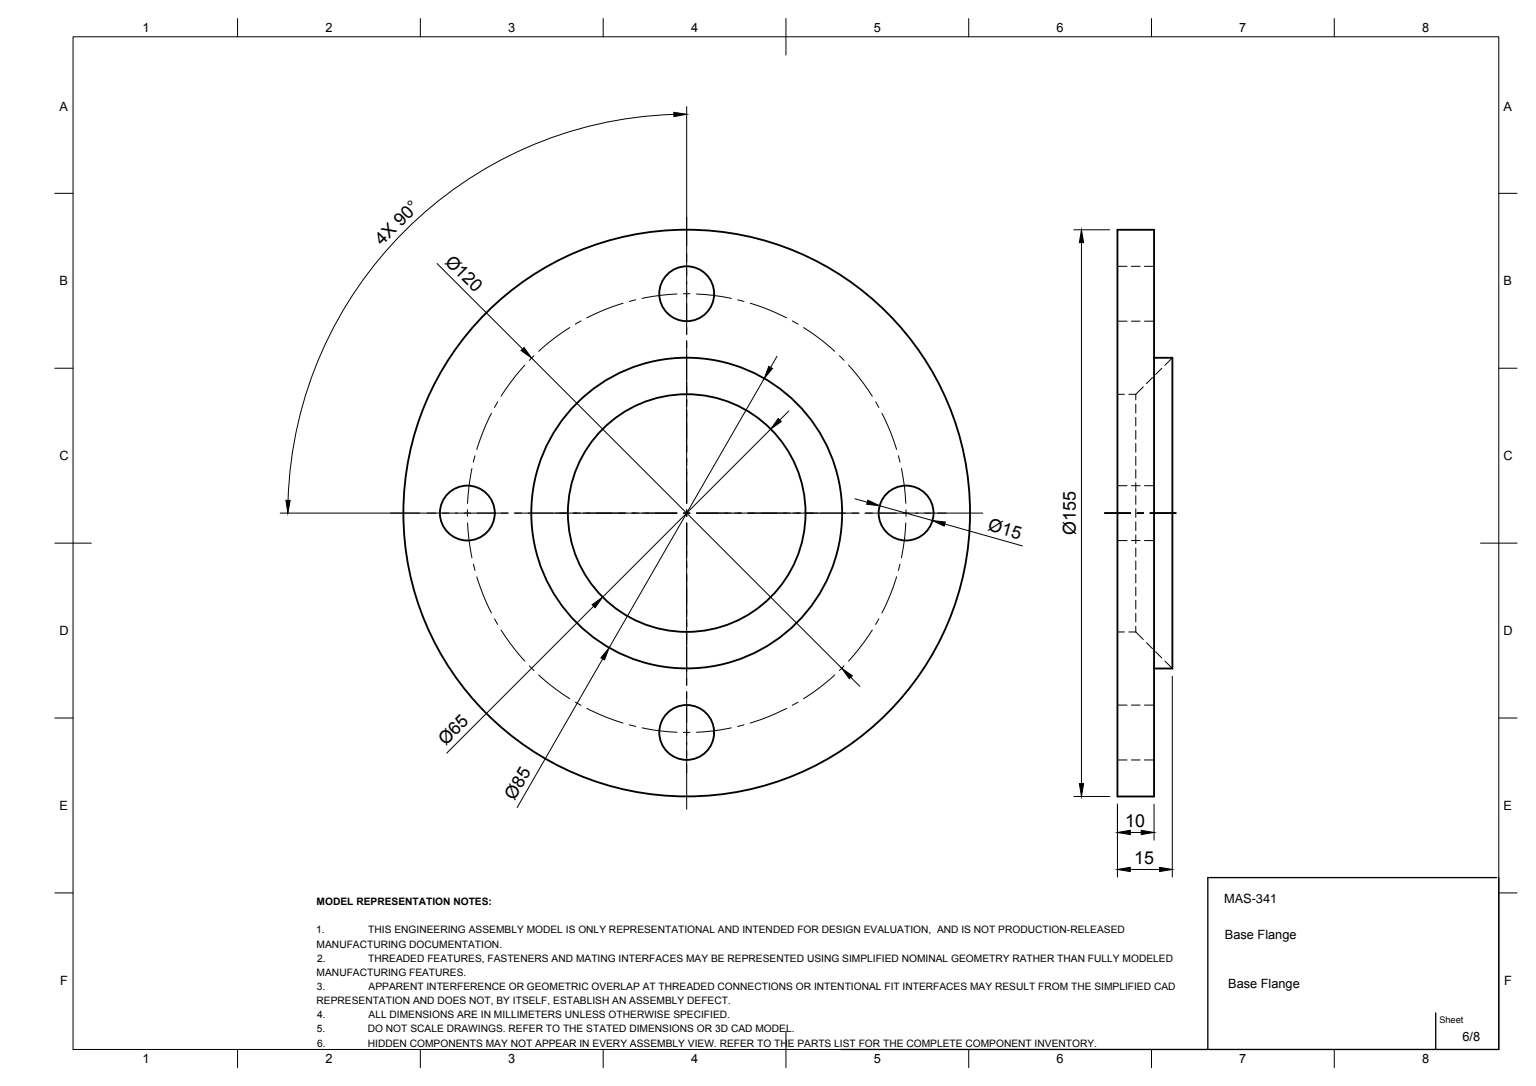
ISO-10303-21;
HEADER;
FILE_DESCRIPTION (('STEP AP214'),
    '1' );
FILE_NAME ('Base Flange.step',
    '2026-10-08T00:39:10',
    ( '' ),
    ( '' ),
    'SwSTEP 2.0',
    'SolidWorks 2025',
    '' );
FILE_SCHEMA (( 'AUTOMOTIVE_DESIGN' ));
ENDSEC;

DATA;
#35=DIRECTION ( 'NONE',  ( -0.000000000000000000, -0.000000000000000000, 1.000000000000000000 ) ) ;
#98=VERTEX_POINT ( 'NONE', #17267 ) ;
#119=ORIENTED_EDGE ( 'NONE', *, *, #13238, .T. ) ;
#143=CIRCLE ( 'NONE', #11572, 77.50000000000000000 ) ;
#167=ORIENTED_EDGE ( 'NONE', *, *, #19754, .F. ) ;
#188=( GEOMETRIC_REPRESENTATION_CONTEXT ( 3 ) GLOBAL_UNCERTAINTY_ASSIGNED_CONTEXT ( ( #9055 ) ) GLOBAL_UNIT_ASSIGNED_CONTEXT ( ( #6659, #405, #9614 ) ) REPRESENTATION_CONTEXT ( 'NONE', 'WORKASPACE' ) );
#215=ORIENTED_EDGE ( 'NONE', *, *, #14623, .F. ) ;
#270=VERTEX_POINT ( 'NONE', #10443 ) ;
#322=EDGE_LOOP ( 'NONE', ( #19155, #18434, #14933, #18302 ) ) ;
#335=DIRECTION ( 'NONE',  ( -0.000000000000000000, -0.000000000000000000, 1.000000000000000000 ) ) ;
#336=DIRECTION ( 'NONE',  ( -0.000000000000000000, -0.000000000000000000, 1.000000000000000000 ) ) ;
#359=CARTESIAN_POINT ( 'NONE',  ( 0.000000000000000000, 0.000000000000000000, -110.0000000000000000 ) ) ;
#405=( NAMED_UNIT ( * ) PLANE_ANGLE_UNIT ( ) SI_UNIT ( $, .RADIAN. ) );
#414=DIRECTION ( 'NONE',  ( 1.000000000000000000, 0.000000000000000000, 0.000000000000000000 ) ) ;
#420=AXIS2_PLACEMENT_3D ( 'NONE', #20059, #15147, #19952 ) ;
#423=CYLINDRICAL_SURFACE ( 'NONE', #14783, 77.50000000000000000 ) ;
#435=DIRECTION ( 'NONE',  ( -1.000000000000000000, 0.000000000000000000, 0.000000000000000000 ) ) ;
#443=CARTESIAN_POINT ( 'NONE',  ( 52.50000000000000711, 6.293851260911244545E-13, -115.0000000000000000 ) ) ;
#482=DIRECTION ( 'NONE',  ( 1.000000000000000000, 0.000000000000000000, 0.000000000000000000 ) ) ;
#529=ORIENTED_EDGE ( 'NONE', *, *, #2169, .T. ) ;
#557=VECTOR ( 'NONE', #16246, 1000.000000000000000 ) ;
#598=VECTOR ( 'NONE', #5827, 1000.000000000000000 ) ;
#610=AXIS2_PLACEMENT_3D ( 'NONE', #18415, #15333, #2864 ) ;
#800=FACE_OUTER_BOUND ( 'NONE', #13112, .T. ) ;
#839=ORIENTED_EDGE ( 'NONE', *, *, #18273, .F. ) ;
#840=ORIENTED_EDGE ( 'NONE', *, *, #17283, .T. ) ;
#862=CLOSED_SHELL ( 'NONE', ( #17922, #12414, #11863, #7855, #11249, #16008, #19643, #18744, #7325, #8273, #4630, #7416, #13850, #8626, #3371, #2282, #10782, #5475 ) ) ;
#1012=EDGE_LOOP ( 'NONE', ( #5410, #2459 ) ) ;
#1023=DIRECTION ( 'NONE',  ( -0.000000000000000000, -0.000000000000000000, 1.000000000000000000 ) ) ;
#1072=FACE_OUTER_BOUND ( 'NONE', #19255, .T. ) ;
#1123=EDGE_CURVE ( 'NONE', #2923, #13175, #17579, .T. ) ;
#1126=CARTESIAN_POINT ( 'NONE',  ( 7.500000000000420997, -60.00000000000000000, -115.0000000000000000 ) ) ;
#1215=AXIS2_PLACEMENT_3D ( 'NONE', #17388, #3363, #5010 ) ;
#1231=DIRECTION ( 'NONE',  ( 0.000000000000000000, 0.000000000000000000, -1.000000000000000000 ) ) ;
#1240=SHAPE_REPRESENTATION_RELATIONSHIP ( 'NONE' , 'NONE' ,  #6269, #19668 ) ;
#1250=FACE_OUTER_BOUND ( 'NONE', #9273, .T. ) ;
#1270=VERTEX_POINT ( 'NONE', #8648 ) ;
#1387=CARTESIAN_POINT ( 'NONE',  ( 60.00000000000000711, 6.284666409917639535E-13, -115.0000000000000000 ) ) ;
#1398=CARTESIAN_POINT ( 'NONE',  ( -42.50000000000000000, 5.204748896376250896E-15, -120.0000000000000142 ) ) ;
#1407=CIRCLE ( 'NONE', #20017, 77.50000000000000000 ) ;
#1423=AXIS2_PLACEMENT_3D ( 'NONE', #17058, #18904, #3048 ) ;
#1484=EDGE_CURVE ( 'NONE', #9791, #19232, #143, .T. ) ;
#1670=CYLINDRICAL_SURFACE ( 'NONE', #7935, 7.500000000000002665 ) ;
#1672=CARTESIAN_POINT ( 'NONE',  ( -60.00000000000000000, -2.094888803305880013E-13, -115.0000000000000000 ) ) ;
#1678=CARTESIAN_POINT ( 'NONE',  ( -60.00000000000000000, -2.094888803305880013E-13, -105.0000000000000142 ) ) ;
#1682=AXIS2_PLACEMENT_3D ( 'NONE', #2629, #13551, #19903 ) ;
#1691=CARTESIAN_POINT ( 'NONE',  ( 77.50000000000000000, 0.000000000000000000, -115.0000000000000000 ) ) ;
#1738=SURFACE_STYLE_USAGE ( .BOTH. , #16167 ) ;
#1823=DIRECTION ( 'NONE',  ( 0.000000000000000000, 0.000000000000000000, -1.000000000000000000 ) ) ;
#1840=FILL_AREA_STYLE_COLOUR ( '', #11290 ) ;
#1885=APPLICATION_CONTEXT ( 'automotive_design' ) ;
#1915=AXIS2_PLACEMENT_3D ( 'NONE', #4817, #9513, #17085 ) ;
#1929=CYLINDRICAL_SURFACE ( 'NONE', #15307, 42.50000000000000000 ) ;
#1932=EDGE_CURVE ( 'NONE', #8191, #1945, #2018, .T. ) ;
#1945=VERTEX_POINT ( 'NONE', #17707 ) ;
#2004=CARTESIAN_POINT ( 'NONE',  ( 32.50000000000000000, 0.000000000000000000, -105.0000000000000142 ) ) ;
#2018=CIRCLE ( 'NONE', #13747, 7.500000000000002665 ) ;
#2030=EDGE_CURVE ( 'NONE', #10487, #3058, #19649, .T. ) ;
#2038=ORIENTED_EDGE ( 'NONE', *, *, #15262, .F. ) ;
#2051=FILL_AREA_STYLE ('',( #1840 ) ) ;
#2060=ORIENTED_EDGE ( 'NONE', *, *, #14600, .T. ) ;
#2113=VERTEX_POINT ( 'NONE', #2877 ) ;
#2131=CARTESIAN_POINT ( 'NONE',  ( 0.000000000000000000, 0.000000000000000000, -120.0000000000000142 ) ) ;
#2155=PRODUCT_DEFINITION_SHAPE ( 'NONE', 'NONE',  #8137 ) ;
#2169=EDGE_CURVE ( 'NONE', #3058, #5289, #19323, .T. ) ;
#2231=DIRECTION ( 'NONE',  ( -1.000000000000000000, 0.000000000000000000, 0.000000000000000000 ) ) ;
#2234=DIRECTION ( 'NONE',  ( -0.000000000000000000, -0.000000000000000000, 1.000000000000000000 ) ) ;
#2239=AXIS2_PLACEMENT_3D ( 'NONE', #7821, #13955, #17557 ) ;
#2260=AXIS2_PLACEMENT_3D ( 'NONE', #3132, #9363, #15295 ) ;
#2282=ADVANCED_FACE ( 'NONE', ( #1072 ), #12016, .F. ) ;
#2439=VERTEX_POINT ( 'NONE', #9052 ) ;
#2459=ORIENTED_EDGE ( 'NONE', *, *, #10492, .T. ) ;
#2474=EDGE_CURVE ( 'NONE', #2923, #5289, #12531, .T. ) ;
#2568=VECTOR ( 'NONE', #7390, 1000.000000000000000 ) ;
#2578=EDGE_CURVE ( 'NONE', #2923, #10487, #15266, .T. ) ;
#2582=AXIS2_PLACEMENT_3D ( 'NONE', #4303, #12172, #10532 ) ;
#2584=CIRCLE ( 'NONE', #12038, 7.500000000000002665 ) ;
#2629=CARTESIAN_POINT ( 'NONE',  ( 60.00000000000000711, 6.284666409917639535E-13, -115.0000000000000000 ) ) ;
#2761=LINE ( 'NONE', #9193, #598 ) ;
#2783=FACE_OUTER_BOUND ( 'NONE', #18255, .T. ) ;
#2842=ORIENTED_EDGE ( 'NONE', *, *, #14623, .T. ) ;
#2859=EDGE_CURVE ( 'NONE', #5289, #19124, #15274, .T. ) ;
#2864=DIRECTION ( 'NONE',  ( -1.000000000000000000, 0.000000000000000000, 0.000000000000000000 ) ) ;
#2877=CARTESIAN_POINT ( 'NONE',  ( 67.50000000000000000, 6.284666409917639535E-13, -115.0000000000000000 ) ) ;
#2897=DIRECTION ( 'NONE',  ( -1.000000000000000000, 0.000000000000000000, 0.000000000000000000 ) ) ;
#2905=DIRECTION ( 'NONE',  ( 0.000000000000000000, 0.000000000000000000, -1.000000000000000000 ) ) ;
#2923=VERTEX_POINT ( 'NONE', #14052 ) ;
#2947=DIRECTION ( 'NONE',  ( 0.000000000000000000, 0.000000000000000000, -1.000000000000000000 ) ) ;
#3006=CARTESIAN_POINT ( 'NONE',  ( -52.50000000000000000, -2.094888803305880013E-13, -105.0000000000000142 ) ) ;
#3048=DIRECTION ( 'NONE',  ( 1.000000000000000000, 0.000000000000000000, 0.000000000000000000 ) ) ;
#3058=VERTEX_POINT ( 'NONE', #12609 ) ;
#3132=CARTESIAN_POINT ( 'NONE',  ( 0.000000000000000000, 60.00000000000000000, -115.0000000000000000 ) ) ;
#3253=CARTESIAN_POINT ( 'NONE',  ( 0.000000000000000000, 60.00000000000000000, -115.0000000000000000 ) ) ;
#3254=CARTESIAN_POINT ( 'NONE',  ( -32.50000000000000000, 3.980102097228898626E-15, -115.0000000000000000 ) ) ;
#3255=DIRECTION ( 'NONE',  ( -0.000000000000000000, -0.000000000000000000, 1.000000000000000000 ) ) ;
#3274=EDGE_CURVE ( 'NONE', #9040, #13775, #11187, .T. ) ;
#3282=CARTESIAN_POINT ( 'NONE',  ( 60.00000000000000711, 6.284666409917639535E-13, -105.0000000000000142 ) ) ;
#3302=EDGE_LOOP ( 'NONE', ( #5917, #12026 ) ) ;
#3309=DIRECTION ( 'NONE',  ( -0.000000000000000000, -0.000000000000000000, 1.000000000000000000 ) ) ;
#3363=DIRECTION ( 'NONE',  ( 0.000000000000000000, 0.000000000000000000, -1.000000000000000000 ) ) ;
#3366=VERTEX_POINT ( 'NONE', #12064 ) ;
#3371=ADVANCED_FACE ( 'NONE', ( #2783 ), #18328, .F. ) ;
#3415=CARTESIAN_POINT ( 'NONE',  ( -7.499999999999583444, -60.00000000000000000, -115.0000000000000000 ) ) ;
#3610=( GEOMETRIC_REPRESENTATION_CONTEXT ( 3 ) GLOBAL_UNCERTAINTY_ASSIGNED_CONTEXT ( ( #6235 ) ) GLOBAL_UNIT_ASSIGNED_CONTEXT ( ( #13510, #5655, #13305 ) ) REPRESENTATION_CONTEXT ( 'NONE', 'WORKASPACE' ) );
#3680=LINE ( 'NONE', #19335, #7385 ) ;
#3860=ORIENTED_EDGE ( 'NONE', *, *, #11561, .T. ) ;
#3878=AXIS2_PLACEMENT_3D ( 'NONE', #3253, #2947, #4577 ) ;
#3966=CARTESIAN_POINT ( 'NONE',  ( 0.000000000000000000, 0.000000000000000000, -105.0000000000000142 ) ) ;
#3982=LINE ( 'NONE', #5332, #13486 ) ;
#4004=EDGE_CURVE ( 'NONE', #270, #19664, #12961, .T. ) ;
#4039=EDGE_CURVE ( 'NONE', #19664, #12482, #11515, .T. ) ;
#4199=CIRCLE ( 'NONE', #2260, 7.500000000000001776 ) ;
#4201=LINE ( 'NONE', #1126, #17785 ) ;
#4202=FACE_BOUND ( 'NONE', #16039, .T. ) ;
#4224=AXIS2_PLACEMENT_3D ( 'NONE', #16878, #18420, #7360 ) ;
#4267=DIRECTION ( 'NONE',  ( 1.000000000000000000, 0.000000000000000000, 0.000000000000000000 ) ) ;
#4301=FACE_BOUND ( 'NONE', #11309, .T. ) ;
#4303=CARTESIAN_POINT ( 'NONE',  ( 4.189777606611760026E-13, -60.00000000000000000, -115.0000000000000000 ) ) ;
#4432=CARTESIAN_POINT ( 'NONE',  ( 0.000000000000000000, 0.000000000000000000, -110.0000000000000000 ) ) ;
#4452=DIRECTION ( 'NONE',  ( -1.000000000000000000, 0.000000000000000000, 0.000000000000000000 ) ) ;
#4520=AXIS2_PLACEMENT_3D ( 'NONE', #5919, #18089, #4267 ) ;
#4577=DIRECTION ( 'NONE',  ( -1.000000000000000000, 0.000000000000000000, 0.000000000000000000 ) ) ;
#4630=ADVANCED_FACE ( 'NONE', ( #16080 ), #423, .T. ) ;
#4663=AXIS2_PLACEMENT_3D ( 'NONE', #16689, #1231, #12170 ) ;
#4694=EDGE_LOOP ( 'NONE', ( #12069, #3860 ) ) ;
#4736=EDGE_CURVE ( 'NONE', #9040, #10253, #3982, .T. ) ;
#4781=ORIENTED_EDGE ( 'NONE', *, *, #2859, .F. ) ;
#4793=EDGE_LOOP ( 'NONE', ( #840, #13871, #13576, #16723 ) ) ;
#4817=CARTESIAN_POINT ( 'NONE',  ( 0.000000000000000000, 0.000000000000000000, -115.0000000000000000 ) ) ;
#4844=ORIENTED_EDGE ( 'NONE', *, *, #2578, .T. ) ;
#4948=DIRECTION ( 'NONE',  ( -1.000000000000000000, 0.000000000000000000, 0.000000000000000000 ) ) ;
#4987=EDGE_LOOP ( 'NONE', ( #7887, #4844, #12073, #17622 ) ) ;
#4996=CYLINDRICAL_SURFACE ( 'NONE', #13636, 42.50000000000000000 ) ;
#5010=DIRECTION ( 'NONE',  ( -1.000000000000000000, 0.000000000000000000, 0.000000000000000000 ) ) ;
#5027=DIRECTION ( 'NONE',  ( 0.000000000000000000, 0.000000000000000000, -1.000000000000000000 ) ) ;
#5143=DIRECTION ( 'NONE',  ( 1.000000000000000000, 0.000000000000000000, 0.000000000000000000 ) ) ;
#5205=FACE_OUTER_BOUND ( 'NONE', #9961, .T. ) ;
#5238=CARTESIAN_POINT ( 'NONE',  ( 0.000000000000000000, 0.000000000000000000, -110.0000000000000000 ) ) ;
#5289=VERTEX_POINT ( 'NONE', #1398 ) ;
#5332=CARTESIAN_POINT ( 'NONE',  ( -52.50000000000000000, -2.094888803305880013E-13, -115.0000000000000000 ) ) ;
#5335=ORIENTED_EDGE ( 'NONE', *, *, #16859, .F. ) ;
#5347=ORIENTED_EDGE ( 'NONE', *, *, #13140, .F. ) ;
#5410=ORIENTED_EDGE ( 'NONE', *, *, #11477, .T. ) ;
#5429=DIRECTION ( 'NONE',  ( 1.000000000000000000, 0.000000000000000000, 0.000000000000000000 ) ) ;
#5475=ADVANCED_FACE ( 'NONE', ( #17122 ), #9658, .F. ) ;
#5476=AXIS2_PLACEMENT_3D ( 'NONE', #359, #9672, #11412 ) ;
#5507=CARTESIAN_POINT ( 'NONE',  ( 0.000000000000000000, 0.000000000000000000, -105.0000000000000142 ) ) ;
#5512=DIRECTION ( 'NONE',  ( -1.000000000000000000, 0.000000000000000000, -0.000000000000000000 ) ) ;
#5600=ORIENTED_EDGE ( 'NONE', *, *, #1484, .F. ) ;
#5642=CARTESIAN_POINT ( 'NONE',  ( 32.50000000000000000, 3.980102097228898626E-15, -110.0000000000000000 ) ) ;
#5655=( NAMED_UNIT ( * ) PLANE_ANGLE_UNIT ( ) SI_UNIT ( $, .RADIAN. ) );
#5678=APPLICATION_CONTEXT ( 'automotive_design' ) ;
#5703=VERTEX_POINT ( 'NONE', #19994 ) ;
#5716=DIRECTION ( 'NONE',  ( -1.000000000000000000, 0.000000000000000000, 0.000000000000000000 ) ) ;
#5754=VECTOR ( 'NONE', #1023, 1000.000000000000000 ) ;
#5827=DIRECTION ( 'NONE',  ( -0.000000000000000000, -0.000000000000000000, 1.000000000000000000 ) ) ;
#5917=ORIENTED_EDGE ( 'NONE', *, *, #11967, .F. ) ;
#5919=CARTESIAN_POINT ( 'NONE',  ( 60.00000000000000711, 6.284666409917639535E-13, -115.0000000000000000 ) ) ;
#5929=DIRECTION ( 'NONE',  ( 0.000000000000000000, 0.000000000000000000, -1.000000000000000000 ) ) ;
#5947=CARTESIAN_POINT ( 'NONE',  ( -7.499999999999583444, -60.00000000000000000, -105.0000000000000142 ) ) ;
#5950=DIRECTION ( 'NONE',  ( 0.7071067811865493491, 8.659560562354956277E-17, -0.7071067811865455743 ) ) ;
#5951=FACE_BOUND ( 'NONE', #3302, .T. ) ;
#6013=ORIENTED_EDGE ( 'NONE', *, *, #4039, .F. ) ;
#6045=EDGE_CURVE ( 'NONE', #19232, #9109, #3680, .T. ) ;
#6048=ORIENTED_EDGE ( 'NONE', *, *, #2030, .F. ) ;
#6128=VECTOR ( 'NONE', #7701, 1000.000000000000000 ) ;
#6200=ORIENTED_EDGE ( 'NONE', *, *, #2169, .F. ) ;
#6202=CIRCLE ( 'NONE', #12388, 42.50000000000000000 ) ;
#6216=CIRCLE ( 'NONE', #16012, 77.50000000000000000 ) ;
#6235=UNCERTAINTY_MEASURE_WITH_UNIT (LENGTH_MEASURE( 1.000000000000000082E-05 ), #13510, 'distance_accuracy_value', 'NONE');
#6258=EDGE_CURVE ( 'NONE', #3366, #10253, #15903, .T. ) ;
#6269=SHAPE_REPRESENTATION ( 'Base Flange', ( #18639 ), #3610 ) ;
#6352=VECTOR ( 'NONE', #335, 1000.000000000000000 ) ;
#6385=CIRCLE ( 'NONE', #16822, 7.500000000000002665 ) ;
#6435=AXIS2_PLACEMENT_3D ( 'NONE', #17070, #13783, #15427 ) ;
#6515=CARTESIAN_POINT ( 'NONE',  ( -60.00000000000000000, -2.094888803305880013E-13, -115.0000000000000000 ) ) ;
#6523=EDGE_CURVE ( 'NONE', #2113, #98, #18073, .T. ) ;
#6619=ORIENTED_EDGE ( 'NONE', *, *, #12893, .T. ) ;
#6659=( LENGTH_UNIT ( ) NAMED_UNIT ( * ) SI_UNIT ( .MILLI., .METRE. ) );
#6662=EDGE_CURVE ( 'NONE', #16938, #2113, #13773, .T. ) ;
#6664=AXIS2_PLACEMENT_3D ( 'NONE', #11876, #10549, #2897 ) ;
#6674=DIRECTION ( 'NONE',  ( -0.000000000000000000, -0.000000000000000000, 1.000000000000000000 ) ) ;
#6711=FACE_OUTER_BOUND ( 'NONE', #15002, .T. ) ;
#6725=CARTESIAN_POINT ( 'NONE',  ( 0.000000000000000000, 0.000000000000000000, -120.0000000000000142 ) ) ;
#6802=VERTEX_POINT ( 'NONE', #2004 ) ;
#6850=VECTOR ( 'NONE', #17659, 1000.000000000000000 ) ;
#6911=CYLINDRICAL_SURFACE ( 'NONE', #8795, 7.500000000000000000 ) ;
#7004=EDGE_CURVE ( 'NONE', #16938, #19717, #9550, .T. ) ;
#7033=EDGE_CURVE ( 'NONE', #5703, #8191, #19074, .T. ) ;
#7049=FACE_BOUND ( 'NONE', #20046, .T. ) ;
#7165=DIRECTION ( 'NONE',  ( -0.000000000000000000, -0.000000000000000000, 1.000000000000000000 ) ) ;
#7205=CARTESIAN_POINT ( 'NONE',  ( 0.000000000000000000, 60.00000000000000000, -105.0000000000000142 ) ) ;
#7325=ADVANCED_FACE ( 'NONE', ( #13708, #18326, #15243, #5951, #4301, #4202 ), #10432, .T. ) ;
#7339=FACE_BOUND ( 'NONE', #12467, .T. ) ;
#7360=DIRECTION ( 'NONE',  ( -1.000000000000000000, 0.000000000000000000, 0.000000000000000000 ) ) ;
#7365=LINE ( 'NONE', #10734, #5754 ) ;
#7385=VECTOR ( 'NONE', #35, 1000.000000000000000 ) ;
#7390=DIRECTION ( 'NONE',  ( -0.000000000000000000, -0.000000000000000000, 1.000000000000000000 ) ) ;
#7416=ADVANCED_FACE ( 'NONE', ( #9423 ), #18842, .F. ) ;
#7517=ORIENTED_EDGE ( 'NONE', *, *, #6258, .F. ) ;
#7521=PRODUCT_DEFINITION_FORMATION_WITH_SPECIFIED_SOURCE ( 'ANY', '', #9652, .NOT_KNOWN. ) ;
#7537=CIRCLE ( 'NONE', #8203, 7.500000000000001776 ) ;
#7630=ORIENTED_EDGE ( 'NONE', *, *, #4736, .T. ) ;
#7701=DIRECTION ( 'NONE',  ( -0.000000000000000000, -0.000000000000000000, 1.000000000000000000 ) ) ;
#7712=DIRECTION ( 'NONE',  ( 0.000000000000000000, 0.000000000000000000, -1.000000000000000000 ) ) ;
#7718=ORIENTED_EDGE ( 'NONE', *, *, #6258, .T. ) ;
#7721=DIRECTION ( 'NONE',  ( 0.000000000000000000, 0.000000000000000000, -1.000000000000000000 ) ) ;
#7793=EDGE_LOOP ( 'NONE', ( #13389, #19862, #529, #19927 ) ) ;
#7821=CARTESIAN_POINT ( 'NONE',  ( 0.000000000000000000, 0.000000000000000000, -115.0000000000000000 ) ) ;
#7855=ADVANCED_FACE ( 'NONE', ( #1250 ), #1670, .F. ) ;
#7887=ORIENTED_EDGE ( 'NONE', *, *, #1123, .F. ) ;
#7909=ORIENTED_EDGE ( 'NONE', *, *, #11561, .F. ) ;
#7935=AXIS2_PLACEMENT_3D ( 'NONE', #10652, #3309, #17222 ) ;
#7980=ORIENTED_EDGE ( 'NONE', *, *, #6662, .F. ) ;
#8002=DIRECTION ( 'NONE',  ( -0.000000000000000000, -0.000000000000000000, 1.000000000000000000 ) ) ;
#8016=EDGE_CURVE ( 'NONE', #2113, #16938, #9255, .T. ) ;
#8137=PRODUCT_DEFINITION ( 'UNKNOWN', '', #7521, #17854 ) ;
#8158=DIRECTION ( 'NONE',  ( -0.000000000000000000, -0.000000000000000000, 1.000000000000000000 ) ) ;
#8191=VERTEX_POINT ( 'NONE', #5947 ) ;
#8195=ORIENTED_EDGE ( 'NONE', *, *, #2474, .T. ) ;
#8197=PRODUCT_CONTEXT ( 'NONE', #1885, 'mechanical' ) ;
#8202=ORIENTED_EDGE ( 'NONE', *, *, #18273, .T. ) ;
#8203=AXIS2_PLACEMENT_3D ( 'NONE', #7205, #16424, #8831 ) ;
#8228=MANIFOLD_SOLID_BREP ( 'Chamfer2', #862 ) ;
#8238=ORIENTED_EDGE ( 'NONE', *, *, #6045, .F. ) ;
#8273=ADVANCED_FACE ( 'NONE', ( #800, #13167, #7049, #7339, #8478, #10015 ), #11826, .F. ) ;
#8294=ORIENTED_EDGE ( 'NONE', *, *, #8997, .F. ) ;
#8416=CARTESIAN_POINT ( 'NONE',  ( 0.000000000000000000, 0.000000000000000000, 0.000000000000000000 ) ) ;
#8478=FACE_BOUND ( 'NONE', #14442, .T. ) ;
#8509=ORIENTED_EDGE ( 'NONE', *, *, #4039, .T. ) ;
#8525=ORIENTED_EDGE ( 'NONE', *, *, #14166, .T. ) ;
#8599=EDGE_LOOP ( 'NONE', ( #17999, #17197, #5335, #14175 ) ) ;
#8626=ADVANCED_FACE ( 'NONE', ( #15690 ), #12705, .F. ) ;
#8631=DIRECTION ( 'NONE',  ( 1.000000000000000000, 0.000000000000000000, 0.000000000000000000 ) ) ;
#8648=CARTESIAN_POINT ( 'NONE',  ( 7.500000000000001776, 60.00000000000000000, -115.0000000000000000 ) ) ;
#8771=EDGE_CURVE ( 'NONE', #10487, #6802, #7365, .T. ) ;
#8791=DIRECTION ( 'NONE',  ( -0.000000000000000000, -0.000000000000000000, 1.000000000000000000 ) ) ;
#8795=AXIS2_PLACEMENT_3D ( 'NONE', #6515, #12734, #9224 ) ;
#8831=DIRECTION ( 'NONE',  ( -1.000000000000000000, 0.000000000000000000, 0.000000000000000000 ) ) ;
#8880=CYLINDRICAL_SURFACE ( 'NONE', #16105, 7.500000000000001776 ) ;
#8997=EDGE_CURVE ( 'NONE', #19717, #98, #14222, .T. ) ;
#9040=VERTEX_POINT ( 'NONE', #9917 ) ;
#9052=CARTESIAN_POINT ( 'NONE',  ( 42.50000000000000000, 0.000000000000000000, -115.0000000000000000 ) ) ;
#9055=UNCERTAINTY_MEASURE_WITH_UNIT (LENGTH_MEASURE( 1.000000000000000082E-05 ), #6659, 'distance_accuracy_value', 'NONE');
#9097=ORIENTED_EDGE ( 'NONE', *, *, #7004, .F. ) ;
#9109=VERTEX_POINT ( 'NONE', #10016 ) ;
#9127=CARTESIAN_POINT ( 'NONE',  ( -32.50000000000000000, 3.980102097228898626E-15, -105.0000000000000142 ) ) ;
#9129=CIRCLE ( 'NONE', #1915, 77.50000000000000000 ) ;
#9133=DIRECTION ( 'NONE',  ( -1.000000000000000000, 0.000000000000000000, 0.000000000000000000 ) ) ;
#9193=CARTESIAN_POINT ( 'NONE',  ( 7.500000000000001776, 60.00000000000000000, -115.0000000000000000 ) ) ;
#9224=DIRECTION ( 'NONE',  ( 1.000000000000000000, 0.000000000000000000, 0.000000000000000000 ) ) ;
#9255=CIRCLE ( 'NONE', #12843, 7.500000000000000000 ) ;
#9273=EDGE_LOOP ( 'NONE', ( #15004, #10275, #15041, #215 ) ) ;
#9347=ORIENTED_EDGE ( 'NONE', *, *, #13519, .F. ) ;
#9363=DIRECTION ( 'NONE',  ( 0.000000000000000000, 0.000000000000000000, -1.000000000000000000 ) ) ;
#9400=ORIENTED_EDGE ( 'NONE', *, *, #20142, .T. ) ;
#9423=FACE_OUTER_BOUND ( 'NONE', #4987, .T. ) ;
#9462=CIRCLE ( 'NONE', #9781, 42.50000000000000000 ) ;
#9473=CARTESIAN_POINT ( 'NONE',  ( -32.50000000000000000, 0.000000000000000000, -110.0000000000000000 ) ) ;
#9513=DIRECTION ( 'NONE',  ( 0.000000000000000000, 0.000000000000000000, -1.000000000000000000 ) ) ;
#9550=LINE ( 'NONE', #443, #14449 ) ;
#9614=( NAMED_UNIT ( * ) SI_UNIT ( $, .STERADIAN. ) SOLID_ANGLE_UNIT ( ) );
#9633=EDGE_LOOP ( 'NONE', ( #15613, #18021 ) ) ;
#9646=DIRECTION ( 'NONE',  ( -0.000000000000000000, -0.000000000000000000, 1.000000000000000000 ) ) ;
#9652=PRODUCT ( 'Base Flange', 'Base Flange', '', ( #8197 ) ) ;
#9658=CONICAL_SURFACE ( 'NONE', #9981, 32.50000000000000000, 0.7853981633974510546 ) ;
#9661=CARTESIAN_POINT ( 'NONE',  ( 0.000000000000000000, 0.000000000000000000, -115.0000000000000000 ) ) ;
#9672=DIRECTION ( 'NONE',  ( 0.000000000000000000, 0.000000000000000000, -1.000000000000000000 ) ) ;
#9725=DIRECTION ( 'NONE',  ( 0.000000000000000000, 0.000000000000000000, -1.000000000000000000 ) ) ;
#9726=CARTESIAN_POINT ( 'NONE',  ( 0.000000000000000000, 0.000000000000000000, -115.0000000000000000 ) ) ;
#9745=DIRECTION ( 'NONE',  ( 0.000000000000000000, 0.000000000000000000, -1.000000000000000000 ) ) ;
#9763=LINE ( 'NONE', #14673, #6850 ) ;
#9781=AXIS2_PLACEMENT_3D ( 'NONE', #18963, #14242, #4948 ) ;
#9791=VERTEX_POINT ( 'NONE', #1691 ) ;
#9861=EDGE_CURVE ( 'NONE', #5289, #3058, #6202, .T. ) ;
#9868=CARTESIAN_POINT ( 'NONE',  ( 0.000000000000000000, 0.000000000000000000, -115.0000000000000000 ) ) ;
#9905=EDGE_CURVE ( 'NONE', #3058, #2439, #9763, .T. ) ;
#9917=CARTESIAN_POINT ( 'NONE',  ( -52.50000000000000000, -2.094888803305880013E-13, -115.0000000000000000 ) ) ;
#9936=SHAPE_DEFINITION_REPRESENTATION ( #2155, #6269 ) ;
#9943=DIRECTION ( 'NONE',  ( 0.000000000000000000, 0.000000000000000000, -1.000000000000000000 ) ) ;
#9961=EDGE_LOOP ( 'NONE', ( #4781, #6200, #18126, #6619 ) ) ;
#9981=AXIS2_PLACEMENT_3D ( 'NONE', #4432, #2905, #9133 ) ;
#10015=FACE_BOUND ( 'NONE', #9633, .T. ) ;
#10016=CARTESIAN_POINT ( 'NONE',  ( -77.50000000000000000, 9.491012693391988181E-15, -105.0000000000000142 ) ) ;
#10069=FACE_OUTER_BOUND ( 'NONE', #12669, .T. ) ;
#10098=DIRECTION ( 'NONE',  ( 1.000000000000000000, 0.000000000000000000, 0.000000000000000000 ) ) ;
#10102=CARTESIAN_POINT ( 'NONE',  ( -7.500000000000001776, 60.00000000000000000, -115.0000000000000000 ) ) ;
#10128=CARTESIAN_POINT ( 'NONE',  ( 60.00000000000000711, 6.284666409917639535E-13, -105.0000000000000142 ) ) ;
#10144=EDGE_CURVE ( 'NONE', #17054, #9109, #6216, .T. ) ;
#10166=CYLINDRICAL_SURFACE ( 'NONE', #17631, 77.50000000000000000 ) ;
#10248=VECTOR ( 'NONE', #11323, 1000.000000000000000 ) ;
#10253=VERTEX_POINT ( 'NONE', #3006 ) ;
#10275=ORIENTED_EDGE ( 'NONE', *, *, #7033, .T. ) ;
#10306=CARTESIAN_POINT ( 'NONE',  ( 32.50000000000000000, 0.000000000000000000, -110.0000000000000000 ) ) ;
#10325=ORIENTED_EDGE ( 'NONE', *, *, #20142, .F. ) ;
#10432=PLANE ( 'NONE',  #4663 ) ;
#10443=CARTESIAN_POINT ( 'NONE',  ( -7.500000000000001776, 60.00000000000000000, -115.0000000000000000 ) ) ;
#10469=AXIS2_PLACEMENT_3D ( 'NONE', #14603, #1823, #16143 ) ;
#10487=VERTEX_POINT ( 'NONE', #10306 ) ;
#10490=ORIENTED_EDGE ( 'NONE', *, *, #6662, .T. ) ;
#10492=EDGE_CURVE ( 'NONE', #13175, #6802, #14971, .T. ) ;
#10532=DIRECTION ( 'NONE',  ( 1.000000000000000000, 0.000000000000000000, 0.000000000000000000 ) ) ;
#10549=DIRECTION ( 'NONE',  ( 0.000000000000000000, 0.000000000000000000, -1.000000000000000000 ) ) ;
#10564=CARTESIAN_POINT ( 'NONE',  ( 0.000000000000000000, 60.00000000000000000, -105.0000000000000142 ) ) ;
#10605=DIRECTION ( 'NONE',  ( -1.000000000000000000, 0.000000000000000000, 0.000000000000000000 ) ) ;
#10640=ORIENTED_EDGE ( 'NONE', *, *, #13519, .T. ) ;
#10652=CARTESIAN_POINT ( 'NONE',  ( 4.189777606611760026E-13, -60.00000000000000000, -115.0000000000000000 ) ) ;
#10681=ORIENTED_EDGE ( 'NONE', *, *, #4004, .T. ) ;
#10734=CARTESIAN_POINT ( 'NONE',  ( 32.50000000000000000, 0.000000000000000000, -115.0000000000000000 ) ) ;
#10737=EDGE_CURVE ( 'NONE', #5703, #13232, #2584, .T. ) ;
#10782=ADVANCED_FACE ( 'NONE', ( #5205 ), #1929, .T. ) ;
#10895=DIRECTION ( 'NONE',  ( -0.7071067811865493491, 0.000000000000000000, -0.7071067811865455743 ) ) ;
#10930=AXIS2_PLACEMENT_3D ( 'NONE', #1672, #8002, #17437 ) ;
#10944=CARTESIAN_POINT ( 'NONE',  ( 0.000000000000000000, 0.000000000000000000, -115.0000000000000000 ) ) ;
#11063=AXIS2_PLACEMENT_3D ( 'NONE', #13681, #16567, #5716 ) ;
#11107=ORIENTED_EDGE ( 'NONE', *, *, #1932, .T. ) ;
#11187=CIRCLE ( 'NONE', #420, 7.500000000000007105 ) ;
#11249=ADVANCED_FACE ( 'NONE', ( #6711 ), #6911, .F. ) ;
#11290=COLOUR_RGB ( '', 0.09019608, 0.27058824, 0.51372549) ;
#11306=DIRECTION ( 'NONE',  ( 1.000000000000000000, 0.000000000000000000, 0.000000000000000000 ) ) ;
#11308=EDGE_CURVE ( 'NONE', #19124, #2439, #9462, .T. ) ;
#11309=EDGE_LOOP ( 'NONE', ( #2038, #12984 ) ) ;
#11323=DIRECTION ( 'NONE',  ( -0.000000000000000000, -0.000000000000000000, 1.000000000000000000 ) ) ;
#11411=CYLINDRICAL_SURFACE ( 'NONE', #14072, 32.50000000000000000 ) ;
#11412=DIRECTION ( 'NONE',  ( -1.000000000000000000, 0.000000000000000000, 0.000000000000000000 ) ) ;
#11477=EDGE_CURVE ( 'NONE', #6802, #13175, #13044, .T. ) ;
#11515=CIRCLE ( 'NONE', #18051, 7.500000000000001776 ) ;
#11516=AXIS2_PLACEMENT_3D ( 'NONE', #10944, #12475, #414 ) ;
#11561=EDGE_CURVE ( 'NONE', #19232, #9791, #9129, .T. ) ;
#11572=AXIS2_PLACEMENT_3D ( 'NONE', #9661, #7712, #18988 ) ;
#11623=DIRECTION ( 'NONE',  ( 0.000000000000000000, 0.000000000000000000, -1.000000000000000000 ) ) ;
#11729=DIRECTION ( 'NONE',  ( 0.000000000000000000, 0.000000000000000000, -1.000000000000000000 ) ) ;
#11747=CARTESIAN_POINT ( 'NONE',  ( 0.000000000000000000, 60.00000000000000000, -115.0000000000000000 ) ) ;
#11826=PLANE ( 'NONE',  #12920 ) ;
#11863=ADVANCED_FACE ( 'NONE', ( #19710 ), #19812, .F. ) ;
#11876=CARTESIAN_POINT ( 'NONE',  ( -60.00000000000000000, -2.094888803305880013E-13, -115.0000000000000000 ) ) ;
#11925=DIRECTION ( 'NONE',  ( 0.000000000000000000, 0.000000000000000000, -1.000000000000000000 ) ) ;
#11945=CARTESIAN_POINT ( 'NONE',  ( 7.500000000000420997, -60.00000000000000000, -115.0000000000000000 ) ) ;
#11967=EDGE_CURVE ( 'NONE', #1270, #270, #16311, .T. ) ;
#11973=ORIENTED_EDGE ( 'NONE', *, *, #7033, .F. ) ;
#12016=CYLINDRICAL_SURFACE ( 'NONE', #1682, 7.500000000000000000 ) ;
#12026=ORIENTED_EDGE ( 'NONE', *, *, #18508, .F. ) ;
#12038=AXIS2_PLACEMENT_3D ( 'NONE', #12451, #11623, #2231 ) ;
#12064=CARTESIAN_POINT ( 'NONE',  ( -67.50000000000000000, -2.085703952312275003E-13, -105.0000000000000142 ) ) ;
#12069=ORIENTED_EDGE ( 'NONE', *, *, #1484, .T. ) ;
#12073=ORIENTED_EDGE ( 'NONE', *, *, #8771, .T. ) ;
#12085=EDGE_LOOP ( 'NONE', ( #15156, #7980 ) ) ;
#12170=DIRECTION ( 'NONE',  ( -1.000000000000000000, 0.000000000000000000, -0.000000000000000000 ) ) ;
#12172=DIRECTION ( 'NONE',  ( -0.000000000000000000, -0.000000000000000000, 1.000000000000000000 ) ) ;
#12240=EDGE_LOOP ( 'NONE', ( #8238, #5600, #2060, #14237 ) ) ;
#12296=LINE ( 'NONE', #19669, #2568 ) ;
#12388=AXIS2_PLACEMENT_3D ( 'NONE', #18886, #12424, #14066 ) ;
#12414=ADVANCED_FACE ( 'NONE', ( #14089 ), #4996, .T. ) ;
#12424=DIRECTION ( 'NONE',  ( 0.000000000000000000, 0.000000000000000000, -1.000000000000000000 ) ) ;
#12451=CARTESIAN_POINT ( 'NONE',  ( 4.189777606611760026E-13, -60.00000000000000000, -115.0000000000000000 ) ) ;
#12467=EDGE_LOOP ( 'NONE', ( #9400, #7718 ) ) ;
#12470=VECTOR ( 'NONE', #9646, 1000.000000000000000 ) ;
#12475=DIRECTION ( 'NONE',  ( -0.000000000000000000, -0.000000000000000000, 1.000000000000000000 ) ) ;
#12482=VERTEX_POINT ( 'NONE', #13340 ) ;
#12509=DIRECTION ( 'NONE',  ( -1.000000000000000000, 0.000000000000000000, 0.000000000000000000 ) ) ;
#12531=LINE ( 'NONE', #9473, #15381 ) ;
#12609=CARTESIAN_POINT ( 'NONE',  ( 42.50000000000000000, 0.000000000000000000, -120.0000000000000142 ) ) ;
#12641=AXIS2_PLACEMENT_3D ( 'NONE', #10128, #19248, #12987 ) ;
#12644=FACE_OUTER_BOUND ( 'NONE', #13185, .T. ) ;
#12669=EDGE_LOOP ( 'NONE', ( #7909, #12721, #10640, #15075 ) ) ;
#12694=ORIENTED_EDGE ( 'NONE', *, *, #4736, .F. ) ;
#12705=CYLINDRICAL_SURFACE ( 'NONE', #10930, 7.500000000000000000 ) ;
#12721=ORIENTED_EDGE ( 'NONE', *, *, #6045, .T. ) ;
#12734=DIRECTION ( 'NONE',  ( -0.000000000000000000, -0.000000000000000000, 1.000000000000000000 ) ) ;
#12735=CARTESIAN_POINT ( 'NONE',  ( -7.500000000000001776, 60.00000000000000000, -105.0000000000000142 ) ) ;
#12739=CIRCLE ( 'NONE', #15347, 7.500000000000007105 ) ;
#12746=CYLINDRICAL_SURFACE ( 'NONE', #1423, 7.500000000000001776 ) ;
#12834=DIRECTION ( 'NONE',  ( -0.000000000000000000, -0.000000000000000000, 1.000000000000000000 ) ) ;
#12843=AXIS2_PLACEMENT_3D ( 'NONE', #19356, #9943, #435 ) ;
#12883=CARTESIAN_POINT ( 'NONE',  ( 4.189777606611760026E-13, -60.00000000000000000, -105.0000000000000142 ) ) ;
#12893=EDGE_CURVE ( 'NONE', #2439, #19124, #19861, .T. ) ;
#12920=AXIS2_PLACEMENT_3D ( 'NONE', #3966, #11925, #5512 ) ;
#12934=FACE_OUTER_BOUND ( 'NONE', #4793, .T. ) ;
#12961=LINE ( 'NONE', #10102, #13787 ) ;
#12980=DIRECTION ( 'NONE',  ( -1.000000000000000000, 0.000000000000000000, 0.000000000000000000 ) ) ;
#12984=ORIENTED_EDGE ( 'NONE', *, *, #10737, .F. ) ;
#12987=DIRECTION ( 'NONE',  ( -1.000000000000000000, 0.000000000000000000, 0.000000000000000000 ) ) ;
#13016=ORIENTED_EDGE ( 'NONE', *, *, #3274, .T. ) ;
#13044=CIRCLE ( 'NONE', #4224, 32.50000000000000000 ) ;
#13107=ORIENTED_EDGE ( 'NONE', *, *, #19754, .T. ) ;
#13112=EDGE_LOOP ( 'NONE', ( #16516, #9347 ) ) ;
#13140=EDGE_CURVE ( 'NONE', #13775, #3366, #12296, .T. ) ;
#13156=ORIENTED_EDGE ( 'NONE', *, *, #18508, .T. ) ;
#13167=FACE_BOUND ( 'NONE', #1012, .T. ) ;
#13175=VERTEX_POINT ( 'NONE', #9127 ) ;
#13185=EDGE_LOOP ( 'NONE', ( #18311, #13156, #8202, #6013 ) ) ;
#13221=CARTESIAN_POINT ( 'NONE',  ( 0.000000000000000000, 0.000000000000000000, -115.0000000000000000 ) ) ;
#13229=ORIENTED_EDGE ( 'NONE', *, *, #13140, .T. ) ;
#13232=VERTEX_POINT ( 'NONE', #11945 ) ;
#13238=EDGE_CURVE ( 'NONE', #1945, #8191, #13324, .T. ) ;
#13305=( NAMED_UNIT ( * ) SI_UNIT ( $, .STERADIAN. ) SOLID_ANGLE_UNIT ( ) );
#13324=CIRCLE ( 'NONE', #610, 7.500000000000002665 ) ;
#13340=CARTESIAN_POINT ( 'NONE',  ( 7.500000000000001776, 60.00000000000000000, -105.0000000000000142 ) ) ;
#13389=ORIENTED_EDGE ( 'NONE', *, *, #17283, .F. ) ;
#13486=VECTOR ( 'NONE', #8791, 1000.000000000000000 ) ;
#13500=DIRECTION ( 'NONE',  ( 1.000000000000000000, 0.000000000000000000, 0.000000000000000000 ) ) ;
#13510=( LENGTH_UNIT ( ) NAMED_UNIT ( * ) SI_UNIT ( .MILLI., .METRE. ) );
#13519=EDGE_CURVE ( 'NONE', #9109, #17054, #1407, .T. ) ;
#13536=ORIENTED_EDGE ( 'NONE', *, *, #2578, .F. ) ;
#13551=DIRECTION ( 'NONE',  ( -0.000000000000000000, -0.000000000000000000, 1.000000000000000000 ) ) ;
#13576=ORIENTED_EDGE ( 'NONE', *, *, #11477, .F. ) ;
#13599=CARTESIAN_POINT ( 'NONE',  ( -42.50000000000000000, 5.204748896376250896E-15, -115.0000000000000000 ) ) ;
#13636=AXIS2_PLACEMENT_3D ( 'NONE', #6725, #3255, #482 ) ;
#13654=CONICAL_SURFACE ( 'NONE', #14332, 32.50000000000000000, 0.7853981633974510546 ) ;
#13681=CARTESIAN_POINT ( 'NONE',  ( 0.000000000000000000, 0.000000000000000000, -105.0000000000000142 ) ) ;
#13708=FACE_BOUND ( 'NONE', #12085, .T. ) ;
#13747=AXIS2_PLACEMENT_3D ( 'NONE', #12883, #5027, #12980 ) ;
#13773=CIRCLE ( 'NONE', #14772, 7.500000000000000000 ) ;
#13775=VERTEX_POINT ( 'NONE', #15829 ) ;
#13783=DIRECTION ( 'NONE',  ( 0.000000000000000000, 0.000000000000000000, -1.000000000000000000 ) ) ;
#13787=VECTOR ( 'NONE', #2234, 1000.000000000000000 ) ;
#13796=EDGE_LOOP ( 'NONE', ( #5347, #8525, #7630, #7517 ) ) ;
#13850=ADVANCED_FACE ( 'NONE', ( #12644 ), #12746, .F. ) ;
#13871=ORIENTED_EDGE ( 'NONE', *, *, #1123, .T. ) ;
#13891=CARTESIAN_POINT ( 'NONE',  ( 77.50000000000000000, 0.000000000000000000, -105.0000000000000142 ) ) ;
#13955=DIRECTION ( 'NONE',  ( 0.000000000000000000, 0.000000000000000000, -1.000000000000000000 ) ) ;
#14029=ORIENTED_EDGE ( 'NONE', *, *, #10737, .T. ) ;
#14052=CARTESIAN_POINT ( 'NONE',  ( -32.50000000000000000, 3.980102097228898626E-15, -110.0000000000000000 ) ) ;
#14066=DIRECTION ( 'NONE',  ( -1.000000000000000000, 0.000000000000000000, 0.000000000000000000 ) ) ;
#14072=AXIS2_PLACEMENT_3D ( 'NONE', #9868, #12834, #11306 ) ;
#14089=FACE_OUTER_BOUND ( 'NONE', #322, .T. ) ;
#14157=DIRECTION ( 'NONE',  ( 0.000000000000000000, 0.000000000000000000, -1.000000000000000000 ) ) ;
#14166=EDGE_CURVE ( 'NONE', #13775, #9040, #14808, .T. ) ;
#14175=ORIENTED_EDGE ( 'NONE', *, *, #6523, .F. ) ;
#14222=CIRCLE ( 'NONE', #19456, 7.500000000000000000 ) ;
#14237=ORIENTED_EDGE ( 'NONE', *, *, #10144, .T. ) ;
#14240=STYLED_ITEM ( 'NONE', ( #17403 ), #8228 ) ;
#14242=DIRECTION ( 'NONE',  ( 0.000000000000000000, 0.000000000000000000, -1.000000000000000000 ) ) ;
#14332=AXIS2_PLACEMENT_3D ( 'NONE', #5238, #9725, #17717 ) ;
#14442=EDGE_LOOP ( 'NONE', ( #119, #11107 ) ) ;
#14449=VECTOR ( 'NONE', #336, 1000.000000000000000 ) ;
#14454=LINE ( 'NONE', #15793, #6352 ) ;
#14600=EDGE_CURVE ( 'NONE', #9791, #17054, #14454, .T. ) ;
#14603=CARTESIAN_POINT ( 'NONE',  ( 0.000000000000000000, 0.000000000000000000, -120.0000000000000142 ) ) ;
#14618=CIRCLE ( 'NONE', #1215, 32.50000000000000000 ) ;
#14623=EDGE_CURVE ( 'NONE', #13232, #1945, #4201, .T. ) ;
#14673=CARTESIAN_POINT ( 'NONE',  ( 42.50000000000000000, 0.000000000000000000, -120.0000000000000142 ) ) ;
#14772=AXIS2_PLACEMENT_3D ( 'NONE', #1387, #7721, #4452 ) ;
#14783=AXIS2_PLACEMENT_3D ( 'NONE', #9726, #6674, #5143 ) ;
#14808=CIRCLE ( 'NONE', #6664, 7.500000000000007105 ) ;
#14905=DIRECTION ( 'NONE',  ( -1.000000000000000000, 0.000000000000000000, 0.000000000000000000 ) ) ;
#14933=ORIENTED_EDGE ( 'NONE', *, *, #11308, .T. ) ;
#14971=CIRCLE ( 'NONE', #11063, 32.50000000000000000 ) ;
#14980=ORIENTED_EDGE ( 'NONE', *, *, #3274, .F. ) ;
#15002=EDGE_LOOP ( 'NONE', ( #13016, #13229, #10325, #12694 ) ) ;
#15004=ORIENTED_EDGE ( 'NONE', *, *, #15262, .T. ) ;
#15041=ORIENTED_EDGE ( 'NONE', *, *, #13238, .F. ) ;
#15075=ORIENTED_EDGE ( 'NONE', *, *, #14600, .F. ) ;
#15147=DIRECTION ( 'NONE',  ( 0.000000000000000000, 0.000000000000000000, -1.000000000000000000 ) ) ;
#15156=ORIENTED_EDGE ( 'NONE', *, *, #8016, .F. ) ;
#15173=CARTESIAN_POINT ( 'NONE',  ( -42.50000000000000000, 5.204748896376250896E-15, -120.0000000000000142 ) ) ;
#15243=FACE_OUTER_BOUND ( 'NONE', #4694, .T. ) ;
#15262=EDGE_CURVE ( 'NONE', #13232, #5703, #6385, .T. ) ;
#15266=CIRCLE ( 'NONE', #5476, 32.50000000000000000 ) ;
#15274=LINE ( 'NONE', #15173, #6128 ) ;
#15295=DIRECTION ( 'NONE',  ( -1.000000000000000000, 0.000000000000000000, 0.000000000000000000 ) ) ;
#15307=AXIS2_PLACEMENT_3D ( 'NONE', #2131, #8158, #10098 ) ;
#15333=DIRECTION ( 'NONE',  ( 0.000000000000000000, 0.000000000000000000, -1.000000000000000000 ) ) ;
#15347=AXIS2_PLACEMENT_3D ( 'NONE', #1678, #9745, #17640 ) ;
#15381=VECTOR ( 'NONE', #10895, 1000.000000000000114 ) ;
#15427=DIRECTION ( 'NONE',  ( -1.000000000000000000, 0.000000000000000000, 0.000000000000000000 ) ) ;
#15613=ORIENTED_EDGE ( 'NONE', *, *, #16859, .T. ) ;
#15690=FACE_OUTER_BOUND ( 'NONE', #13796, .T. ) ;
#15756=DIRECTION ( 'NONE',  ( -1.000000000000000000, 0.000000000000000000, 0.000000000000000000 ) ) ;
#15793=CARTESIAN_POINT ( 'NONE',  ( 77.50000000000000000, 0.000000000000000000, -115.0000000000000000 ) ) ;
#15829=CARTESIAN_POINT ( 'NONE',  ( -67.50000000000000000, -2.085703952312275003E-13, -115.0000000000000000 ) ) ;
#15903=CIRCLE ( 'NONE', #6435, 7.500000000000007105 ) ;
#15953=ORIENTED_EDGE ( 'NONE', *, *, #11967, .T. ) ;
#15960=SURFACE_STYLE_FILL_AREA ( #2051 ) ;
#15980=ORIENTED_EDGE ( 'NONE', *, *, #9861, .T. ) ;
#16008=ADVANCED_FACE ( 'NONE', ( #19727 ), #8880, .F. ) ;
#16012=AXIS2_PLACEMENT_3D ( 'NONE', #19671, #16708, #16417 ) ;
#16039=EDGE_LOOP ( 'NONE', ( #19105, #19662 ) ) ;
#16080=FACE_OUTER_BOUND ( 'NONE', #12240, .T. ) ;
#16105=AXIS2_PLACEMENT_3D ( 'NONE', #11747, #7165, #5429 ) ;
#16143=DIRECTION ( 'NONE',  ( -1.000000000000000000, 0.000000000000000000, 0.000000000000000000 ) ) ;
#16167=SURFACE_SIDE_STYLE ('',( #15960 ) ) ;
#16246=DIRECTION ( 'NONE',  ( -0.000000000000000000, -0.000000000000000000, 1.000000000000000000 ) ) ;
#16301=DIRECTION ( 'NONE',  ( -0.000000000000000000, -0.000000000000000000, 1.000000000000000000 ) ) ;
#16311=CIRCLE ( 'NONE', #3878, 7.500000000000001776 ) ;
#16417=DIRECTION ( 'NONE',  ( -1.000000000000000000, 0.000000000000000000, 0.000000000000000000 ) ) ;
#16424=DIRECTION ( 'NONE',  ( 0.000000000000000000, 0.000000000000000000, -1.000000000000000000 ) ) ;
#16516=ORIENTED_EDGE ( 'NONE', *, *, #10144, .F. ) ;
#16542=CARTESIAN_POINT ( 'NONE',  ( 67.50000000000000000, 6.284666409917639535E-13, -115.0000000000000000 ) ) ;
#16567=DIRECTION ( 'NONE',  ( 0.000000000000000000, 0.000000000000000000, -1.000000000000000000 ) ) ;
#16577=ORIENTED_EDGE ( 'NONE', *, *, #1932, .F. ) ;
#16689=CARTESIAN_POINT ( 'NONE',  ( 0.000000000000000000, 0.000000000000000000, -115.0000000000000000 ) ) ;
#16708=DIRECTION ( 'NONE',  ( 0.000000000000000000, 0.000000000000000000, -1.000000000000000000 ) ) ;
#16723=ORIENTED_EDGE ( 'NONE', *, *, #8771, .F. ) ;
#16822=AXIS2_PLACEMENT_3D ( 'NONE', #16864, #5929, #10605 ) ;
#16845=MECHANICAL_DESIGN_GEOMETRIC_PRESENTATION_REPRESENTATION('',(#14240),#188);
#16859=EDGE_CURVE ( 'NONE', #98, #19717, #19184, .T. ) ;
#16864=CARTESIAN_POINT ( 'NONE',  ( 4.189777606611760026E-13, -60.00000000000000000, -115.0000000000000000 ) ) ;
#16878=CARTESIAN_POINT ( 'NONE',  ( 0.000000000000000000, 0.000000000000000000, -105.0000000000000142 ) ) ;
#16938=VERTEX_POINT ( 'NONE', #17909 ) ;
#17039=VECTOR ( 'NONE', #5950, 1000.000000000000114 ) ;
#17054=VERTEX_POINT ( 'NONE', #13891 ) ;
#17058=CARTESIAN_POINT ( 'NONE',  ( 0.000000000000000000, 60.00000000000000000, -115.0000000000000000 ) ) ;
#17070=CARTESIAN_POINT ( 'NONE',  ( -60.00000000000000000, -2.094888803305880013E-13, -105.0000000000000142 ) ) ;
#17085=DIRECTION ( 'NONE',  ( -1.000000000000000000, 0.000000000000000000, 0.000000000000000000 ) ) ;
#17122=FACE_OUTER_BOUND ( 'NONE', #19584, .T. ) ;
#17197=ORIENTED_EDGE ( 'NONE', *, *, #7004, .T. ) ;
#17222=DIRECTION ( 'NONE',  ( 1.000000000000000000, 0.000000000000000000, 0.000000000000000000 ) ) ;
#17267=CARTESIAN_POINT ( 'NONE',  ( 67.50000000000000000, 6.284666409917639535E-13, -105.0000000000000142 ) ) ;
#17283=EDGE_CURVE ( 'NONE', #10487, #2923, #14618, .T. ) ;
#17388=CARTESIAN_POINT ( 'NONE',  ( 0.000000000000000000, 0.000000000000000000, -110.0000000000000000 ) ) ;
#17403=PRESENTATION_STYLE_ASSIGNMENT (( #1738 ) ) ;
#17421=FACE_OUTER_BOUND ( 'NONE', #7793, .T. ) ;
#17437=DIRECTION ( 'NONE',  ( 1.000000000000000000, 0.000000000000000000, 0.000000000000000000 ) ) ;
#17557=DIRECTION ( 'NONE',  ( -1.000000000000000000, 0.000000000000000000, 0.000000000000000000 ) ) ;
#17579=LINE ( 'NONE', #3254, #10248 ) ;
#17622=ORIENTED_EDGE ( 'NONE', *, *, #10492, .F. ) ;
#17631=AXIS2_PLACEMENT_3D ( 'NONE', #13221, #19481, #8631 ) ;
#17640=DIRECTION ( 'NONE',  ( -1.000000000000000000, 0.000000000000000000, 0.000000000000000000 ) ) ;
#17659=DIRECTION ( 'NONE',  ( -0.000000000000000000, -0.000000000000000000, 1.000000000000000000 ) ) ;
#17707=CARTESIAN_POINT ( 'NONE',  ( 7.500000000000420997, -60.00000000000000000, -105.0000000000000142 ) ) ;
#17717=DIRECTION ( 'NONE',  ( -1.000000000000000000, 0.000000000000000000, 0.000000000000000000 ) ) ;
#17785=VECTOR ( 'NONE', #16301, 1000.000000000000000 ) ;
#17854=PRODUCT_DEFINITION_CONTEXT ( 'detailed design', #5678, 'design' ) ;
#17909=CARTESIAN_POINT ( 'NONE',  ( 52.50000000000000711, 6.293851260911244545E-13, -115.0000000000000000 ) ) ;
#17922=ADVANCED_FACE ( 'NONE', ( #17421 ), #13654, .F. ) ;
#17999=ORIENTED_EDGE ( 'NONE', *, *, #8016, .T. ) ;
#18015=EDGE_LOOP ( 'NONE', ( #15953, #10681, #167, #839 ) ) ;
#18021=ORIENTED_EDGE ( 'NONE', *, *, #8997, .T. ) ;
#18031=DIRECTION ( 'NONE',  ( 0.000000000000000000, 0.000000000000000000, 1.000000000000000000 ) ) ;
#18051=AXIS2_PLACEMENT_3D ( 'NONE', #10564, #14157, #12509 ) ;
#18073=LINE ( 'NONE', #16542, #557 ) ;
#18089=DIRECTION ( 'NONE',  ( -0.000000000000000000, -0.000000000000000000, 1.000000000000000000 ) ) ;
#18126=ORIENTED_EDGE ( 'NONE', *, *, #9905, .T. ) ;
#18255=EDGE_LOOP ( 'NONE', ( #11973, #14029, #2842, #16577 ) ) ;
#18273=EDGE_CURVE ( 'NONE', #1270, #12482, #2761, .T. ) ;
#18302=ORIENTED_EDGE ( 'NONE', *, *, #9905, .F. ) ;
#18311=ORIENTED_EDGE ( 'NONE', *, *, #4004, .F. ) ;
#18326=FACE_BOUND ( 'NONE', #18881, .T. ) ;
#18328=CYLINDRICAL_SURFACE ( 'NONE', #2582, 7.500000000000002665 ) ;
#18415=CARTESIAN_POINT ( 'NONE',  ( 4.189777606611760026E-13, -60.00000000000000000, -105.0000000000000142 ) ) ;
#18420=DIRECTION ( 'NONE',  ( 0.000000000000000000, 0.000000000000000000, -1.000000000000000000 ) ) ;
#18434=ORIENTED_EDGE ( 'NONE', *, *, #2859, .T. ) ;
#18508=EDGE_CURVE ( 'NONE', #270, #1270, #4199, .T. ) ;
#18639=AXIS2_PLACEMENT_3D ( 'NONE', #8416, #18031, #13500 ) ;
#18735=CARTESIAN_POINT ( 'NONE',  ( -77.50000000000000000, 9.491012693391988181E-15, -115.0000000000000000 ) ) ;
#18744=ADVANCED_FACE ( 'NONE', ( #10069 ), #10166, .T. ) ;
#18842=CYLINDRICAL_SURFACE ( 'NONE', #11516, 32.50000000000000000 ) ;
#18881=EDGE_LOOP ( 'NONE', ( #14980, #19960 ) ) ;
#18886=CARTESIAN_POINT ( 'NONE',  ( 0.000000000000000000, 0.000000000000000000, -120.0000000000000142 ) ) ;
#18904=DIRECTION ( 'NONE',  ( -0.000000000000000000, -0.000000000000000000, 1.000000000000000000 ) ) ;
#18963=CARTESIAN_POINT ( 'NONE',  ( 0.000000000000000000, 0.000000000000000000, -115.0000000000000000 ) ) ;
#18988=DIRECTION ( 'NONE',  ( -1.000000000000000000, 0.000000000000000000, 0.000000000000000000 ) ) ;
#19040=DIRECTION ( 'NONE',  ( 0.000000000000000000, 0.000000000000000000, -1.000000000000000000 ) ) ;
#19065=ORIENTED_EDGE ( 'NONE', *, *, #6523, .T. ) ;
#19074=LINE ( 'NONE', #3415, #12470 ) ;
#19105=ORIENTED_EDGE ( 'NONE', *, *, #12893, .F. ) ;
#19124=VERTEX_POINT ( 'NONE', #13599 ) ;
#19155=ORIENTED_EDGE ( 'NONE', *, *, #9861, .F. ) ;
#19184=CIRCLE ( 'NONE', #12641, 7.500000000000000000 ) ;
#19232=VERTEX_POINT ( 'NONE', #18735 ) ;
#19248=DIRECTION ( 'NONE',  ( 0.000000000000000000, 0.000000000000000000, -1.000000000000000000 ) ) ;
#19255=EDGE_LOOP ( 'NONE', ( #9097, #10490, #19065, #8294 ) ) ;
#19323=CIRCLE ( 'NONE', #10469, 42.50000000000000000 ) ;
#19335=CARTESIAN_POINT ( 'NONE',  ( -77.50000000000000000, 9.491012693391988181E-15, -115.0000000000000000 ) ) ;
#19356=CARTESIAN_POINT ( 'NONE',  ( 60.00000000000000711, 6.284666409917639535E-13, -115.0000000000000000 ) ) ;
#19391=CARTESIAN_POINT ( 'NONE',  ( 52.50000000000000711, 6.293851260911244545E-13, -105.0000000000000142 ) ) ;
#19456=AXIS2_PLACEMENT_3D ( 'NONE', #3282, #19040, #15756 ) ;
#19481=DIRECTION ( 'NONE',  ( -0.000000000000000000, -0.000000000000000000, 1.000000000000000000 ) ) ;
#19584=EDGE_LOOP ( 'NONE', ( #6048, #13536, #8195, #15980 ) ) ;
#19643=ADVANCED_FACE ( 'NONE', ( #12934 ), #11411, .F. ) ;
#19649=LINE ( 'NONE', #5642, #17039 ) ;
#19662=ORIENTED_EDGE ( 'NONE', *, *, #11308, .F. ) ;
#19664=VERTEX_POINT ( 'NONE', #12735 ) ;
#19668=ADVANCED_BREP_SHAPE_REPRESENTATION ( '', ( #8228, #18639 ), #3610 ) ;
#19669=CARTESIAN_POINT ( 'NONE',  ( -67.50000000000000000, -2.085703952312275003E-13, -115.0000000000000000 ) ) ;
#19671=CARTESIAN_POINT ( 'NONE',  ( 0.000000000000000000, 0.000000000000000000, -105.0000000000000142 ) ) ;
#19710=FACE_OUTER_BOUND ( 'NONE', #8599, .T. ) ;
#19717=VERTEX_POINT ( 'NONE', #19391 ) ;
#19727=FACE_OUTER_BOUND ( 'NONE', #18015, .T. ) ;
#19754=EDGE_CURVE ( 'NONE', #12482, #19664, #7537, .T. ) ;
#19812=CYLINDRICAL_SURFACE ( 'NONE', #4520, 7.500000000000000000 ) ;
#19861=CIRCLE ( 'NONE', #2239, 42.50000000000000000 ) ;
#19862=ORIENTED_EDGE ( 'NONE', *, *, #2030, .T. ) ;
#19903=DIRECTION ( 'NONE',  ( 1.000000000000000000, 0.000000000000000000, 0.000000000000000000 ) ) ;
#19927=ORIENTED_EDGE ( 'NONE', *, *, #2474, .F. ) ;
#19952=DIRECTION ( 'NONE',  ( -1.000000000000000000, 0.000000000000000000, 0.000000000000000000 ) ) ;
#19960=ORIENTED_EDGE ( 'NONE', *, *, #14166, .F. ) ;
#19994=CARTESIAN_POINT ( 'NONE',  ( -7.499999999999583444, -60.00000000000000000, -115.0000000000000000 ) ) ;
#20017=AXIS2_PLACEMENT_3D ( 'NONE', #5507, #11729, #14905 ) ;
#20046=EDGE_LOOP ( 'NONE', ( #13107, #8509 ) ) ;
#20059=CARTESIAN_POINT ( 'NONE',  ( -60.00000000000000000, -2.094888803305880013E-13, -115.0000000000000000 ) ) ;
#20142=EDGE_CURVE ( 'NONE', #10253, #3366, #12739, .T. ) ;
ENDSEC;
END-ISO-10303-21;
